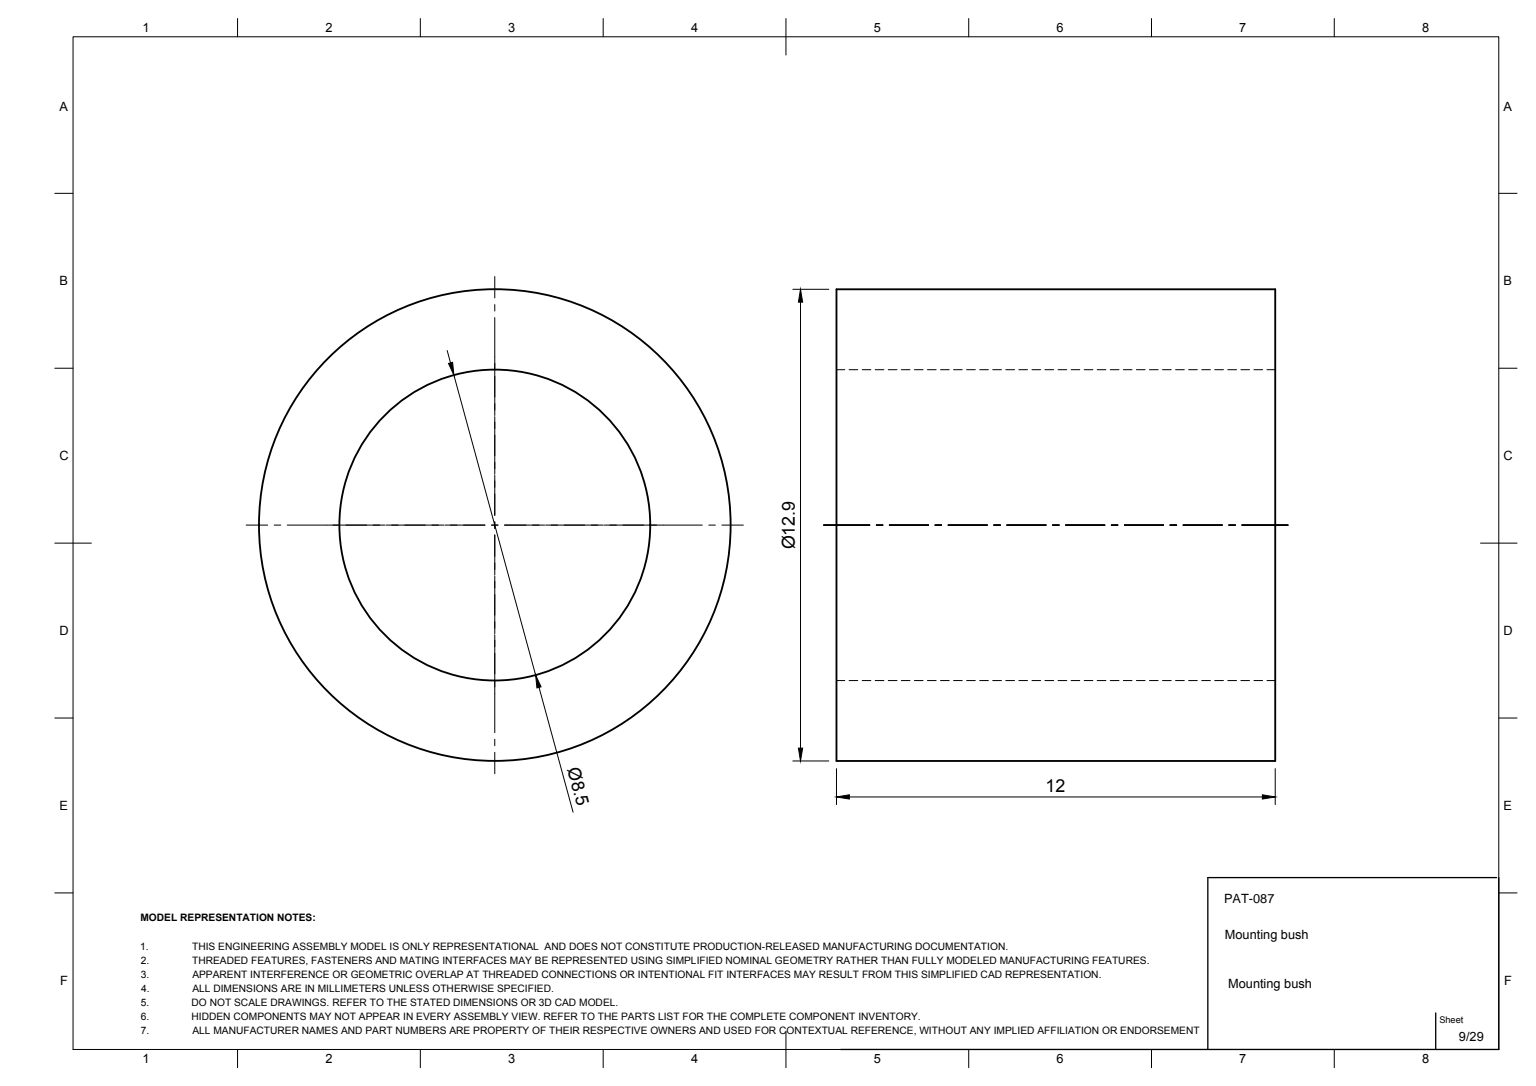
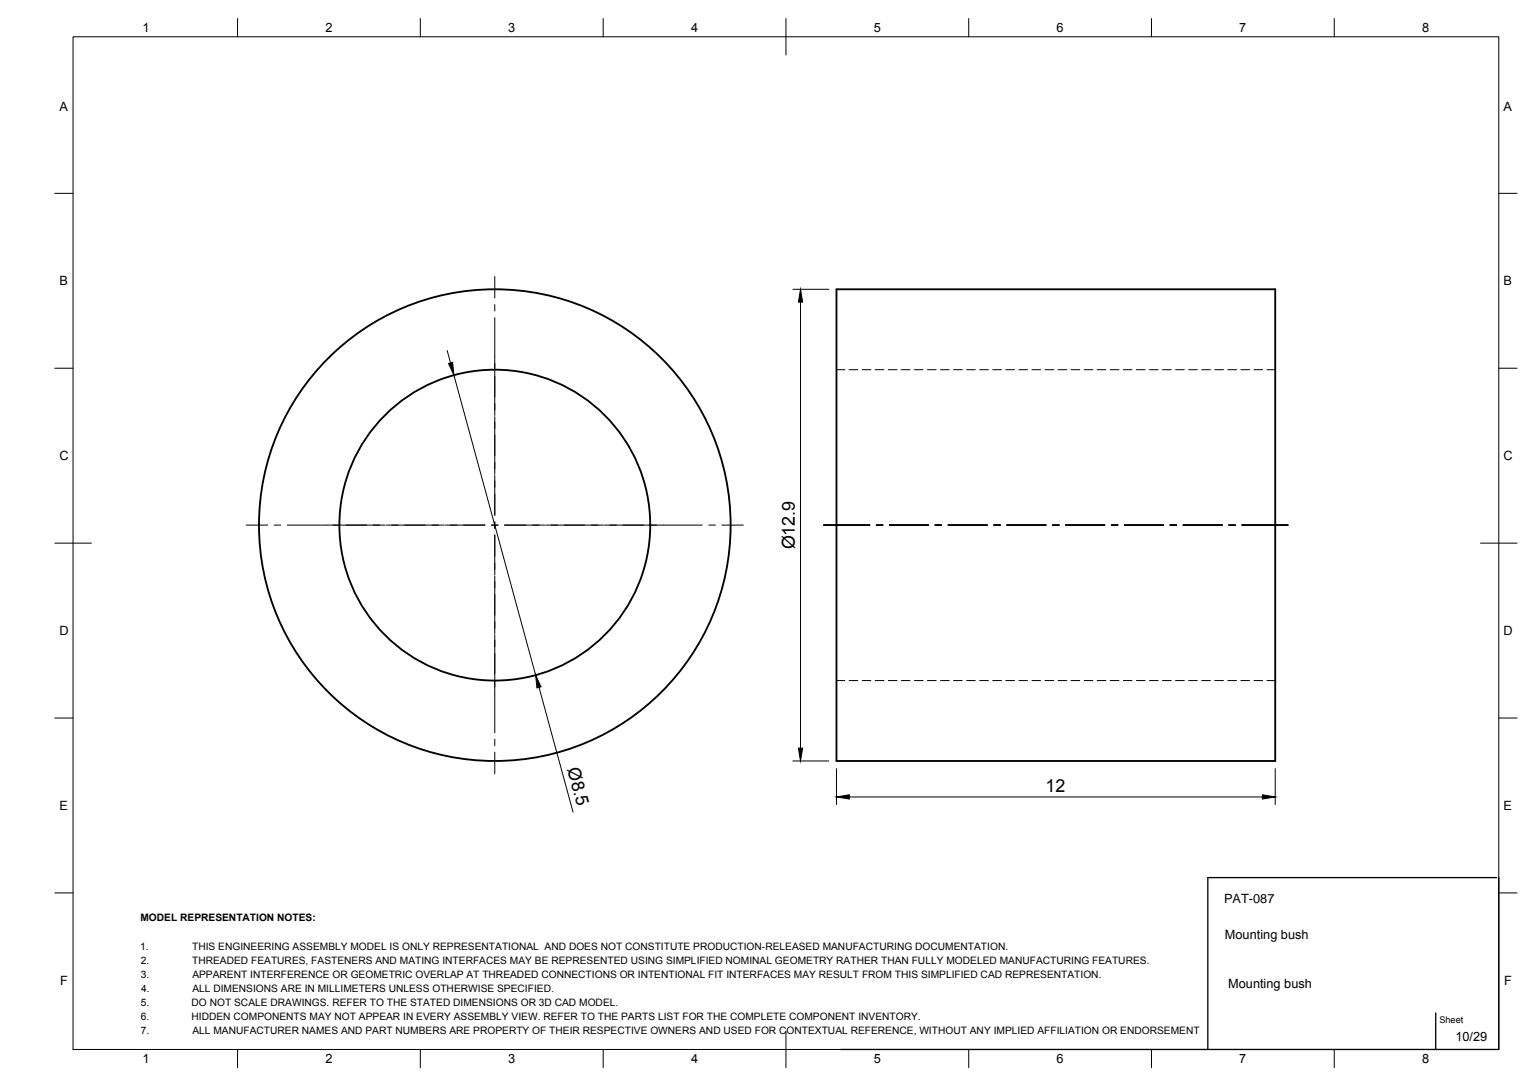
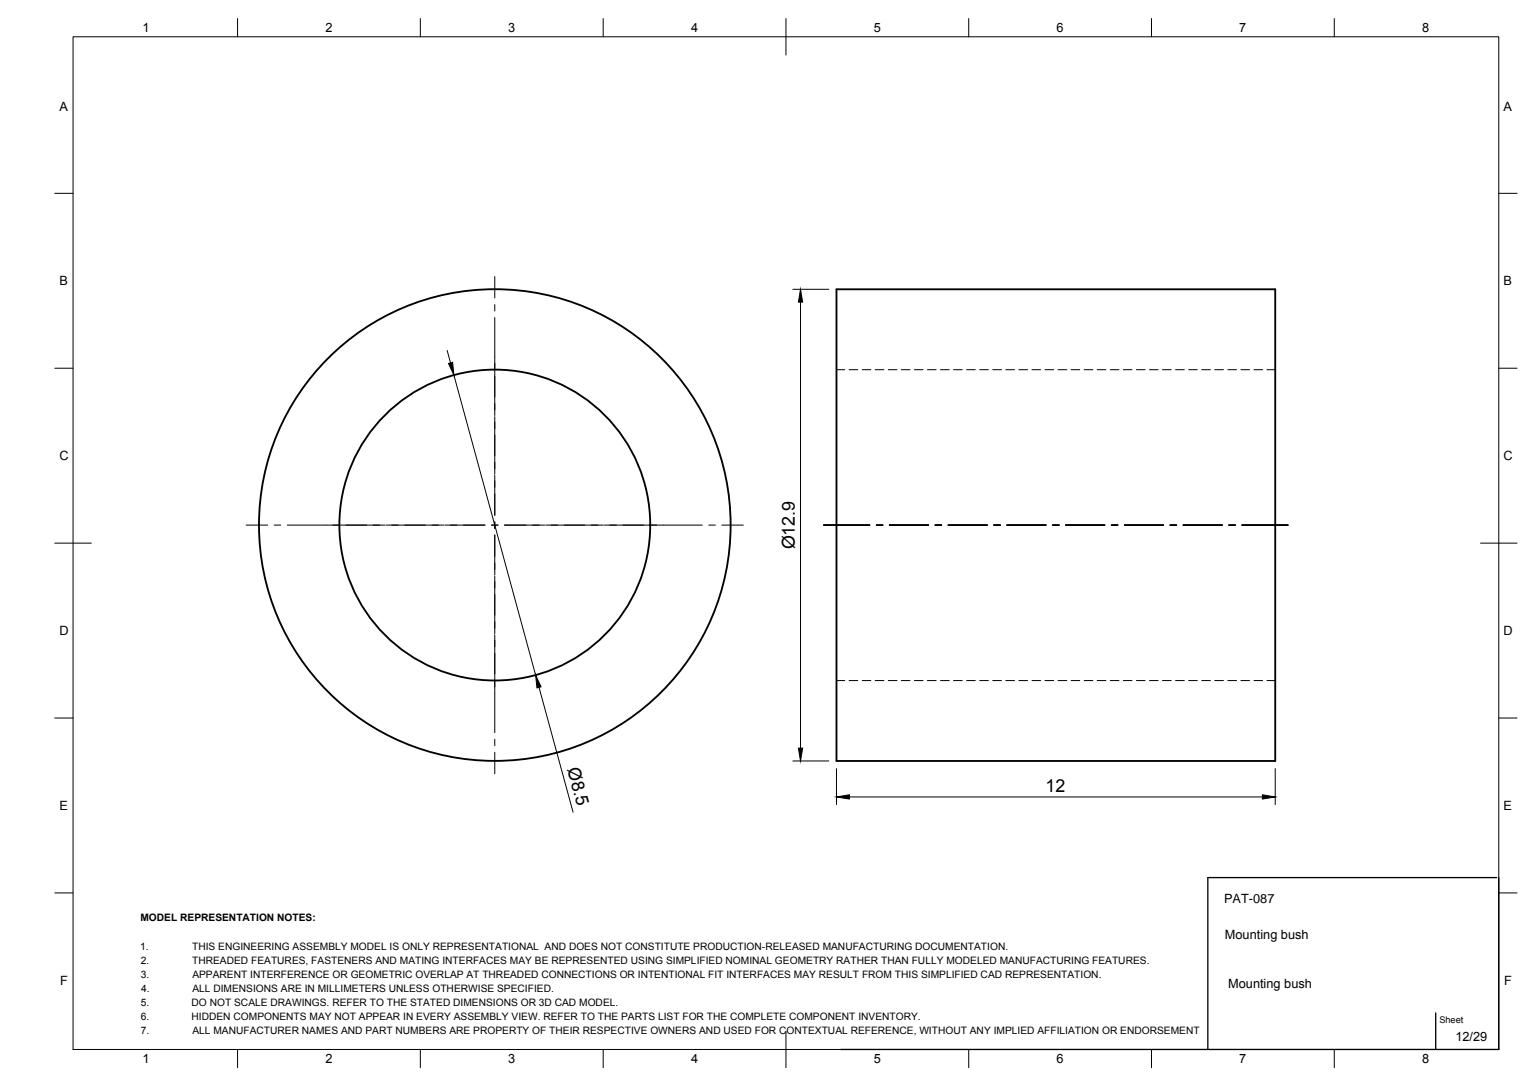
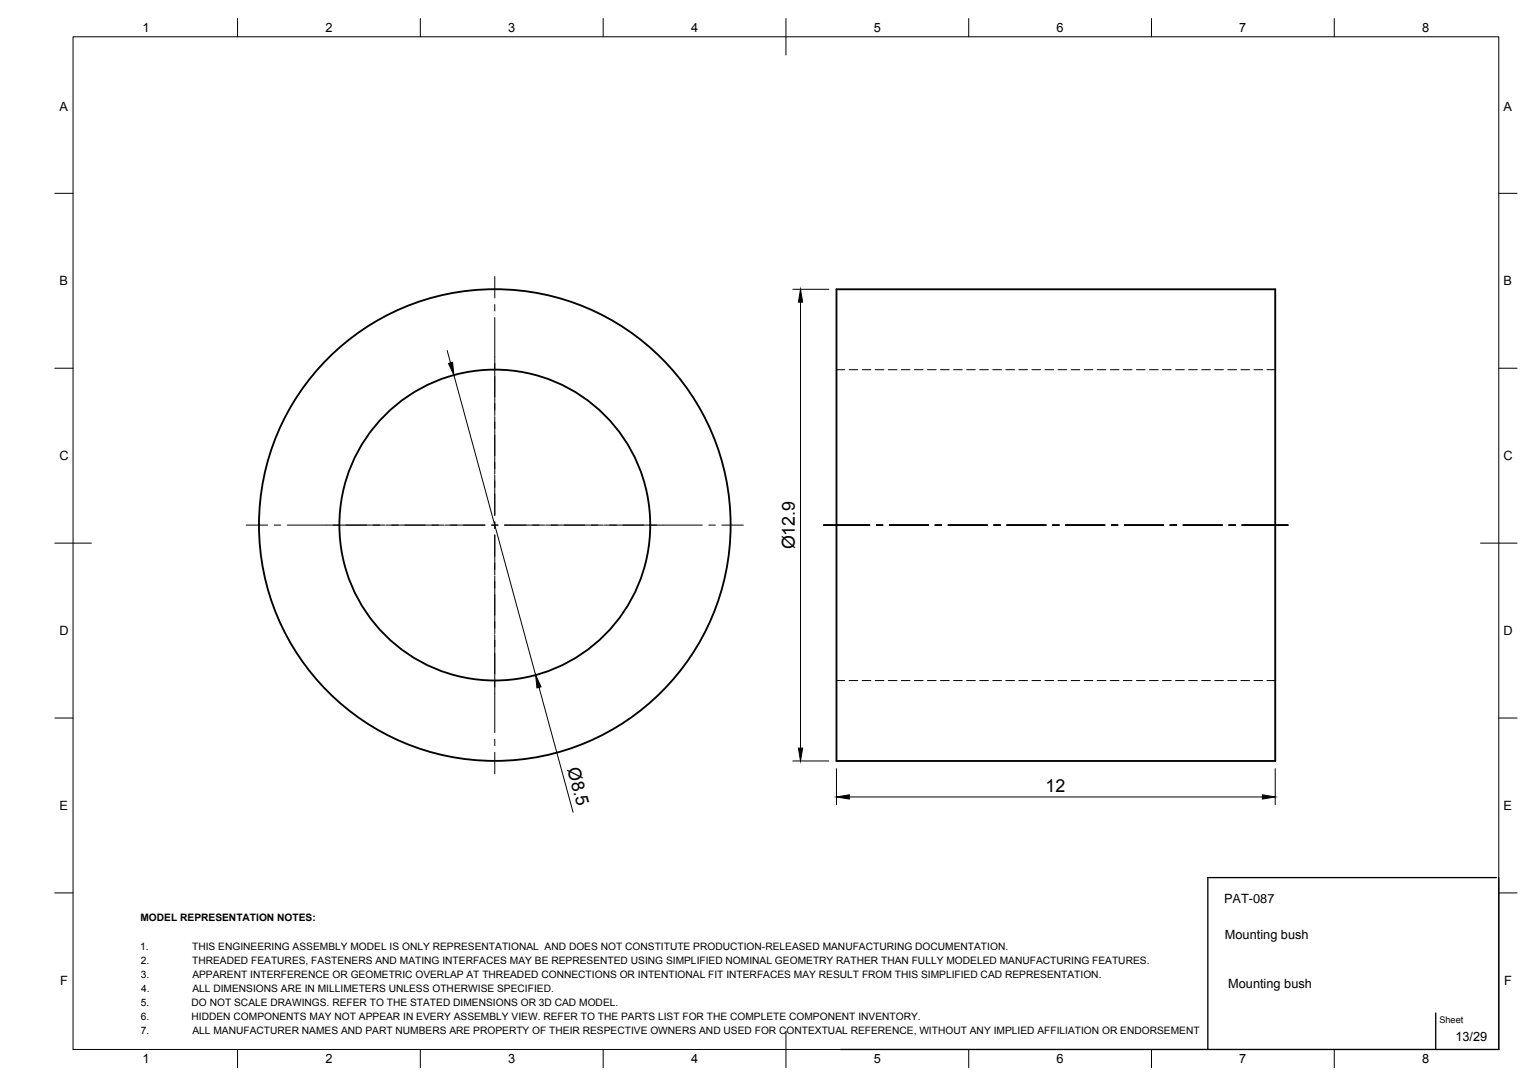
ISO-10303-21;
HEADER;
/* Generated by software containing ST-Developer
 * from STEP Tools, Inc. (www.steptools.com) 
 */

FILE_DESCRIPTION(
/* description */ ('Rigid flange shaft coupling assembly'),
/* implementation_level */ '2;1');

FILE_NAME(
/* name */ 'Mounting bush.step',
/* time_stamp */ '2026-10-27T10:47:16-07:00',
/* author */ (''),
/* organization */ (''),
/* preprocessor_version */ 'ST-DEVELOPER v20.2',
/* originating_system */ 'Autodesk Translation Framework v15.17.0.0',
/* authorisation */ '');

FILE_SCHEMA (('AUTOMOTIVE_DESIGN { 1 0 10303 214 3 1 1 }'));
ENDSEC;

DATA;
#10=MECHANICAL_DESIGN_GEOMETRIC_PRESENTATION_REPRESENTATION('',(#402),#9141);
#346=SHAPE_REPRESENTATION_RELATIONSHIP('SRR','None',#9280,#374);
#374=ADVANCED_BREP_SHAPE_REPRESENTATION('',(#431),#9115);
#402=STYLED_ITEM('',(#9493),#431);
#431=MANIFOLD_SOLID_BREP('Body1',#4756);
#469=FACE_BOUND('',#1067,.T.);
#470=FACE_BOUND('',#1069,.T.);
#594=PLANE('',#5154);
#595=PLANE('',#5155);
#776=FACE_OUTER_BOUND('',#1064,.T.);
#777=FACE_OUTER_BOUND('',#1065,.T.);
#778=FACE_OUTER_BOUND('',#1066,.T.);
#779=FACE_OUTER_BOUND('',#1068,.T.);
#1064=EDGE_LOOP('',(#3387,#3388,#3389,#3390));
#1065=EDGE_LOOP('',(#3391,#3392,#3393,#3394));
#1066=EDGE_LOOP('',(#3395));
#1067=EDGE_LOOP('',(#3396));
#1068=EDGE_LOOP('',(#3397));
#1069=EDGE_LOOP('',(#3398));
#1461=LINE('',#7248,#1806);
#1462=LINE('',#7254,#1807);
#1806=VECTOR('',#5812,0.425);
#1807=VECTOR('',#5819,0.645);
#2111=CIRCLE('',#5149,0.425);
#2112=CIRCLE('',#5150,0.425);
#2113=CIRCLE('',#5152,0.645);
#2114=CIRCLE('',#5153,0.645);
#2324=VERTEX_POINT('',#7245);
#2325=VERTEX_POINT('',#7247);
#2326=VERTEX_POINT('',#7251);
#2327=VERTEX_POINT('',#7253);
#2737=EDGE_CURVE('',#2324,#2324,#2111,.T.);
#2738=EDGE_CURVE('',#2324,#2325,#1461,.T.);
#2739=EDGE_CURVE('',#2325,#2325,#2112,.T.);
#2740=EDGE_CURVE('',#2326,#2326,#2113,.T.);
#2741=EDGE_CURVE('',#2326,#2327,#1462,.T.);
#2742=EDGE_CURVE('',#2327,#2327,#2114,.T.);
#3387=ORIENTED_EDGE('',*,*,#2737,.F.);
#3388=ORIENTED_EDGE('',*,*,#2738,.T.);
#3389=ORIENTED_EDGE('',*,*,#2739,.T.);
#3390=ORIENTED_EDGE('',*,*,#2738,.F.);
#3391=ORIENTED_EDGE('',*,*,#2740,.F.);
#3392=ORIENTED_EDGE('',*,*,#2741,.T.);
#3393=ORIENTED_EDGE('',*,*,#2742,.T.);
#3394=ORIENTED_EDGE('',*,*,#2741,.F.);
#3395=ORIENTED_EDGE('',*,*,#2740,.T.);
#3396=ORIENTED_EDGE('',*,*,#2737,.T.);
#3397=ORIENTED_EDGE('',*,*,#2742,.F.);
#3398=ORIENTED_EDGE('',*,*,#2739,.F.);
#4407=CYLINDRICAL_SURFACE('',#5148,0.425);
#4408=CYLINDRICAL_SURFACE('',#5151,0.645);
#4512=ADVANCED_FACE('',(#776),#4407,.F.);
#4513=ADVANCED_FACE('',(#777),#4408,.T.);
#4514=ADVANCED_FACE('',(#778,#469),#594,.T.);
#4515=ADVANCED_FACE('',(#779,#470),#595,.F.);
#4756=CLOSED_SHELL('',(#4512,#4513,#4514,#4515));
#5147=AXIS2_PLACEMENT_3D('',#7243,#5806,#5807);
#5148=AXIS2_PLACEMENT_3D('',#7244,#5808,#5809);
#5149=AXIS2_PLACEMENT_3D('',#7246,#5810,#5811);
#5150=AXIS2_PLACEMENT_3D('',#7249,#5813,#5814);
#5151=AXIS2_PLACEMENT_3D('',#7250,#5815,#5816);
#5152=AXIS2_PLACEMENT_3D('',#7252,#5817,#5818);
#5153=AXIS2_PLACEMENT_3D('',#7255,#5820,#5821);
#5154=AXIS2_PLACEMENT_3D('',#7256,#5822,#5823);
#5155=AXIS2_PLACEMENT_3D('',#7257,#5824,#5825);
#5806=DIRECTION('axis',(0.,0.,1.));
#5807=DIRECTION('refdir',(1.,0.,0.));
#5808=DIRECTION('center_axis',(0.,0.,1.));
#5809=DIRECTION('ref_axis',(1.,0.,0.));
#5810=DIRECTION('center_axis',(0.,0.,-1.));
#5811=DIRECTION('ref_axis',(1.,0.,0.));
#5812=DIRECTION('',(0.,0.,-1.));
#5813=DIRECTION('center_axis',(0.,0.,-1.));
#5814=DIRECTION('ref_axis',(1.,0.,0.));
#5815=DIRECTION('center_axis',(0.,0.,1.));
#5816=DIRECTION('ref_axis',(1.,0.,0.));
#5817=DIRECTION('center_axis',(0.,0.,1.));
#5818=DIRECTION('ref_axis',(1.,0.,0.));
#5819=DIRECTION('',(0.,0.,-1.));
#5820=DIRECTION('center_axis',(0.,0.,1.));
#5821=DIRECTION('ref_axis',(1.,0.,0.));
#5822=DIRECTION('center_axis',(0.,0.,1.));
#5823=DIRECTION('ref_axis',(1.,0.,0.));
#5824=DIRECTION('center_axis',(0.,0.,1.));
#5825=DIRECTION('ref_axis',(1.,0.,0.));
#7243=CARTESIAN_POINT('',(0.,0.,0.));
#7244=CARTESIAN_POINT('Origin',(-4.75,0.,3.2));
#7245=CARTESIAN_POINT('',(-5.175,-5.20474889637625E-17,4.4));
#7246=CARTESIAN_POINT('Origin',(-4.75,0.,4.4));
#7247=CARTESIAN_POINT('',(-5.175,-5.20474889637625E-17,3.2));
#7248=CARTESIAN_POINT('',(-5.175,-5.20474889637625E-17,3.2));
#7249=CARTESIAN_POINT('Origin',(-4.75,0.,3.2));
#7250=CARTESIAN_POINT('Origin',(-4.75,0.,3.2));
#7251=CARTESIAN_POINT('',(-5.395,-7.89897185450042E-17,4.4));
#7252=CARTESIAN_POINT('Origin',(-4.75,0.,4.4));
#7253=CARTESIAN_POINT('',(-5.395,-7.89897185450042E-17,3.2));
#7254=CARTESIAN_POINT('',(-5.395,-7.89897185450042E-17,3.2));
#7255=CARTESIAN_POINT('Origin',(-4.75,0.,3.2));
#7256=CARTESIAN_POINT('Origin',(-4.75,0.,4.4));
#7257=CARTESIAN_POINT('Origin',(-4.75,0.,3.2));
#9082=UNCERTAINTY_MEASURE_WITH_UNIT(LENGTH_MEASURE(0.001),#9142,
'DISTANCE_ACCURACY_VALUE',
'Maximum model space distance between geometric entities at asserted c
onnectivities');
#9108=UNCERTAINTY_MEASURE_WITH_UNIT(LENGTH_MEASURE(0.001),#9142,
'DISTANCE_ACCURACY_VALUE',
'Maximum model space distance between geometric entities at asserted c
onnectivities');
#9115=(
GEOMETRIC_REPRESENTATION_CONTEXT(3)
GLOBAL_UNCERTAINTY_ASSIGNED_CONTEXT((#9082))
GLOBAL_UNIT_ASSIGNED_CONTEXT((#9142,#9144,#9145))
REPRESENTATION_CONTEXT('','3D')
);
#9141=(
GEOMETRIC_REPRESENTATION_CONTEXT(3)
GLOBAL_UNCERTAINTY_ASSIGNED_CONTEXT((#9108))
GLOBAL_UNIT_ASSIGNED_CONTEXT((#9142,#9144,#9145))
REPRESENTATION_CONTEXT('','3D')
);
#9142=(
LENGTH_UNIT()
NAMED_UNIT(*)
SI_UNIT(.CENTI.,.METRE.)
);
#9144=(
NAMED_UNIT(*)
PLANE_ANGLE_UNIT()
SI_UNIT($,.RADIAN.)
);
#9145=(
NAMED_UNIT(*)
SI_UNIT($,.STERADIAN.)
SOLID_ANGLE_UNIT()
);
#9152=SHAPE_DEFINITION_REPRESENTATION(#9184,#9280);
#9184=PRODUCT_DEFINITION_SHAPE('',$,#9313);
#9280=SHAPE_REPRESENTATION('',(#5147),#9115);
#9306=PRODUCT_DEFINITION_CONTEXT('part definition',#9404,'design');
#9313=PRODUCT_DEFINITION('Mounting bush','Mounting bush',#9345,#9306);
#9345=PRODUCT_DEFINITION_FORMATION('',$,#9412);
#9404=APPLICATION_CONTEXT(
'Core Data for Automotive Mechanical Design Process');
#9405=PRODUCT_CONTEXT('part definition',#9404,'mechanical');
#9412=PRODUCT('Mounting bush','Mounting bush','Mounting bush',(#9405));
#9487=COLOUR_RGB('Sky Blue',0.24,0.69,0.87);
#9488=FILL_AREA_STYLE_COLOUR('',#9487);
#9489=FILL_AREA_STYLE('',(#9488));
#9490=SURFACE_STYLE_FILL_AREA(#9489);
#9491=SURFACE_SIDE_STYLE('',(#9490));
#9492=SURFACE_STYLE_USAGE(.BOTH.,#9491);
#9493=PRESENTATION_STYLE_ASSIGNMENT((#9492));
ENDSEC;
END-ISO-10303-21;
